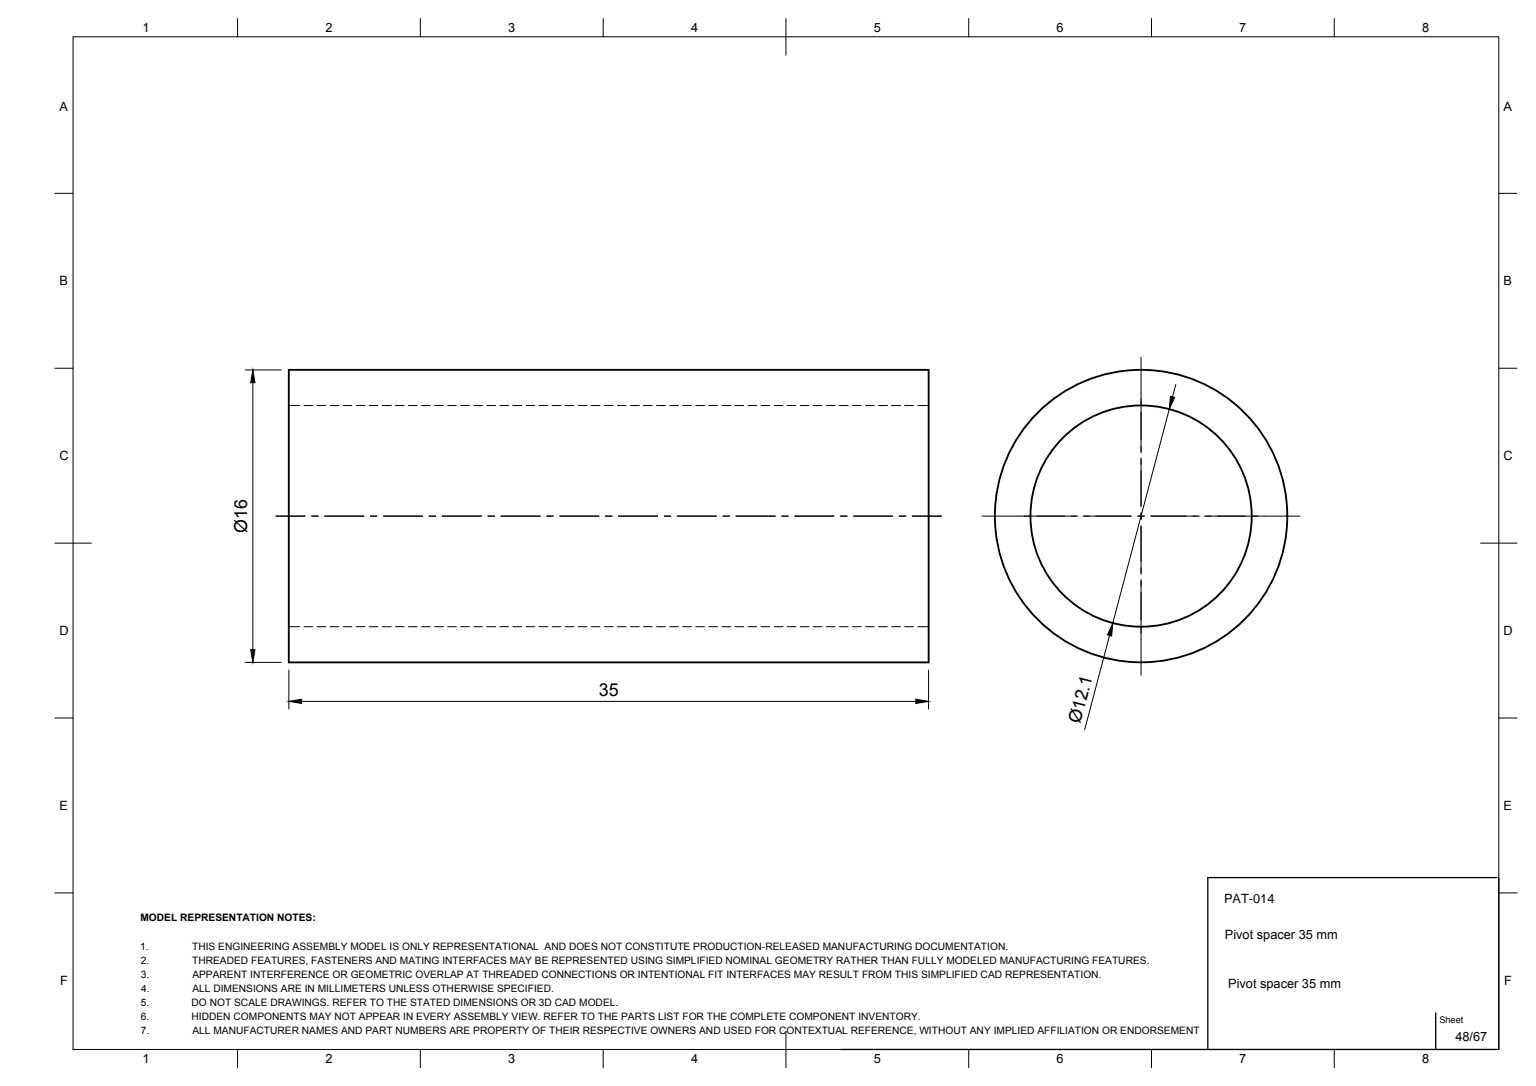
ISO-10303-21;
HEADER;
/* Generated by software containing ST-Developer
 * from STEP Tools, Inc. (www.steptools.com) 
 */

FILE_DESCRIPTION(
/* description */ ('Bin tilter linkage'),
/* implementation_level */ '2;1');

FILE_NAME(
/* name */ 'Pivot spacer 35 mm.step',
/* time_stamp */ '2026-10-28T03:26:24-07:00',
/* author */ (''),
/* organization */ (''),
/* preprocessor_version */ 'ST-DEVELOPER v20.2',
/* originating_system */ 'Autodesk Translation Framework v15.17.0.0',
/* authorisation */ '');

FILE_SCHEMA (('AUTOMOTIVE_DESIGN { 1 0 10303 214 3 1 1 }'));
ENDSEC;

DATA;
#10=MECHANICAL_DESIGN_GEOMETRIC_PRESENTATION_REPRESENTATION('',(#952),#23728);
#732=SHAPE_REPRESENTATION_RELATIONSHIP('SRR','None',#24200,#838);
#838=ADVANCED_BREP_SHAPE_REPRESENTATION('',(#1065),#23700);
#952=STYLED_ITEM('',(#24758),#1065);
#1065=MANIFOLD_SOLID_BREP('Body1',#12483);
#1422=FACE_BOUND('',#3613,.T.);
#1423=FACE_BOUND('',#3615,.T.);
#1788=PLANE('',#15055);
#1789=PLANE('',#15056);
#2498=FACE_OUTER_BOUND('',#3610,.T.);
#2499=FACE_OUTER_BOUND('',#3611,.T.);
#2500=FACE_OUTER_BOUND('',#3612,.T.);
#2501=FACE_OUTER_BOUND('',#3614,.T.);
#3610=EDGE_LOOP('',(#10651,#10652,#10653,#10654));
#3611=EDGE_LOOP('',(#10655,#10656,#10657,#10658));
#3612=EDGE_LOOP('',(#10659));
#3613=EDGE_LOOP('',(#10660));
#3614=EDGE_LOOP('',(#10661));
#3615=EDGE_LOOP('',(#10662));
#4349=LINE('',#22696,#5024);
#4350=LINE('',#22702,#5025);
#5024=VECTOR('',#18724,0.605);
#5025=VECTOR('',#18731,0.800000000000001);
#5824=CIRCLE('',#15050,0.605);
#5825=CIRCLE('',#15051,0.605);
#5826=CIRCLE('',#15053,0.800000000000001);
#5827=CIRCLE('',#15054,0.800000000000001);
#6723=VERTEX_POINT('',#22693);
#6724=VERTEX_POINT('',#22695);
#6725=VERTEX_POINT('',#22699);
#6726=VERTEX_POINT('',#22701);
#8065=EDGE_CURVE('',#6723,#6723,#5824,.T.);
#8066=EDGE_CURVE('',#6723,#6724,#4349,.T.);
#8067=EDGE_CURVE('',#6724,#6724,#5825,.T.);
#8068=EDGE_CURVE('',#6725,#6725,#5826,.T.);
#8069=EDGE_CURVE('',#6725,#6726,#4350,.T.);
#8070=EDGE_CURVE('',#6726,#6726,#5827,.T.);
#10651=ORIENTED_EDGE('',*,*,#8065,.F.);
#10652=ORIENTED_EDGE('',*,*,#8066,.T.);
#10653=ORIENTED_EDGE('',*,*,#8067,.T.);
#10654=ORIENTED_EDGE('',*,*,#8066,.F.);
#10655=ORIENTED_EDGE('',*,*,#8068,.F.);
#10656=ORIENTED_EDGE('',*,*,#8069,.T.);
#10657=ORIENTED_EDGE('',*,*,#8070,.T.);
#10658=ORIENTED_EDGE('',*,*,#8069,.F.);
#10659=ORIENTED_EDGE('',*,*,#8068,.T.);
#10660=ORIENTED_EDGE('',*,*,#8065,.T.);
#10661=ORIENTED_EDGE('',*,*,#8070,.F.);
#10662=ORIENTED_EDGE('',*,*,#8067,.F.);
#11555=CYLINDRICAL_SURFACE('',#15049,0.605);
#11556=CYLINDRICAL_SURFACE('',#15052,0.800000000000001);
#12223=ADVANCED_FACE('',(#2498),#11555,.F.);
#12224=ADVANCED_FACE('',(#2499),#11556,.T.);
#12225=ADVANCED_FACE('',(#2500,#1422),#1788,.T.);
#12226=ADVANCED_FACE('',(#2501,#1423),#1789,.F.);
#12483=CLOSED_SHELL('',(#12223,#12224,#12225,#12226));
#15048=AXIS2_PLACEMENT_3D('',#22691,#18718,#18719);
#15049=AXIS2_PLACEMENT_3D('',#22692,#18720,#18721);
#15050=AXIS2_PLACEMENT_3D('',#22694,#18722,#18723);
#15051=AXIS2_PLACEMENT_3D('',#22697,#18725,#18726);
#15052=AXIS2_PLACEMENT_3D('',#22698,#18727,#18728);
#15053=AXIS2_PLACEMENT_3D('',#22700,#18729,#18730);
#15054=AXIS2_PLACEMENT_3D('',#22703,#18732,#18733);
#15055=AXIS2_PLACEMENT_3D('',#22704,#18734,#18735);
#15056=AXIS2_PLACEMENT_3D('',#22705,#18736,#18737);
#18718=DIRECTION('axis',(0.,0.,1.));
#18719=DIRECTION('refdir',(1.,0.,0.));
#18720=DIRECTION('center_axis',(0.,1.,0.));
#18721=DIRECTION('ref_axis',(1.,0.,0.));
#18722=DIRECTION('center_axis',(0.,-1.,0.));
#18723=DIRECTION('ref_axis',(1.,0.,0.));
#18724=DIRECTION('',(0.,-1.,0.));
#18725=DIRECTION('center_axis',(0.,-1.,0.));
#18726=DIRECTION('ref_axis',(1.,0.,0.));
#18727=DIRECTION('center_axis',(0.,1.,0.));
#18728=DIRECTION('ref_axis',(1.,0.,0.));
#18729=DIRECTION('center_axis',(0.,1.,0.));
#18730=DIRECTION('ref_axis',(1.,0.,0.));
#18731=DIRECTION('',(0.,-1.,0.));
#18732=DIRECTION('center_axis',(0.,1.,0.));
#18733=DIRECTION('ref_axis',(1.,0.,0.));
#18734=DIRECTION('center_axis',(0.,1.,0.));
#18735=DIRECTION('ref_axis',(1.,0.,0.));
#18736=DIRECTION('center_axis',(0.,1.,0.));
#18737=DIRECTION('ref_axis',(1.,0.,0.));
#22691=CARTESIAN_POINT('',(0.,0.,0.));
#22692=CARTESIAN_POINT('Origin',(9.39692620785909,-4.,18.4202014332567));
#22693=CARTESIAN_POINT('',(8.79192620785908,-0.5,18.4202014332567));
#22694=CARTESIAN_POINT('Origin',(9.39692620785909,-0.5,18.4202014332567));
#22695=CARTESIAN_POINT('',(8.79192620785908,-4.,18.4202014332567));
#22696=CARTESIAN_POINT('',(8.79192620785908,-4.,18.4202014332567));
#22697=CARTESIAN_POINT('Origin',(9.39692620785909,-4.,18.4202014332567));
#22698=CARTESIAN_POINT('Origin',(9.39692620785909,-4.,18.4202014332567));
#22699=CARTESIAN_POINT('',(8.59692620785908,-0.5,18.4202014332567));
#22700=CARTESIAN_POINT('Origin',(9.39692620785909,-0.5,18.4202014332567));
#22701=CARTESIAN_POINT('',(8.59692620785908,-4.,18.4202014332567));
#22702=CARTESIAN_POINT('',(8.59692620785908,-4.,18.4202014332567));
#22703=CARTESIAN_POINT('Origin',(9.39692620785909,-4.,18.4202014332567));
#22704=CARTESIAN_POINT('Origin',(9.39692620785909,-0.5,18.4202014332567));
#22705=CARTESIAN_POINT('Origin',(9.39692620785909,-4.,18.4202014332567));
#23583=UNCERTAINTY_MEASURE_WITH_UNIT(LENGTH_MEASURE(0.001),#23729,
'DISTANCE_ACCURACY_VALUE',
'Maximum model space distance between geometric entities at asserted c
onnectivities');
#23611=UNCERTAINTY_MEASURE_WITH_UNIT(LENGTH_MEASURE(0.001),#23729,
'DISTANCE_ACCURACY_VALUE',
'Maximum model space distance between geometric entities at asserted c
onnectivities');
#23700=(
GEOMETRIC_REPRESENTATION_CONTEXT(3)
GLOBAL_UNCERTAINTY_ASSIGNED_CONTEXT((#23583))
GLOBAL_UNIT_ASSIGNED_CONTEXT((#23729,#23731,#23732))
REPRESENTATION_CONTEXT('','3D')
);
#23728=(
GEOMETRIC_REPRESENTATION_CONTEXT(3)
GLOBAL_UNCERTAINTY_ASSIGNED_CONTEXT((#23611))
GLOBAL_UNIT_ASSIGNED_CONTEXT((#23729,#23731,#23732))
REPRESENTATION_CONTEXT('','3D')
);
#23729=(
LENGTH_UNIT()
NAMED_UNIT(*)
SI_UNIT(.CENTI.,.METRE.)
);
#23731=(
NAMED_UNIT(*)
PLANE_ANGLE_UNIT()
SI_UNIT($,.RADIAN.)
);
#23732=(
NAMED_UNIT(*)
SI_UNIT($,.STERADIAN.)
SOLID_ANGLE_UNIT()
);
#23821=SHAPE_DEFINITION_REPRESENTATION(#23988,#24200);
#23988=PRODUCT_DEFINITION_SHAPE('',$,#24317);
#24200=SHAPE_REPRESENTATION('',(#15048),#23700);
#24228=PRODUCT_DEFINITION_CONTEXT('part definition',#24578,'design');
#24317=PRODUCT_DEFINITION('Pivot spacer 35 mm','Pivot spacer 35 mm',#24433,
#24228);
#24433=PRODUCT_DEFINITION_FORMATION('',$,#24668);
#24578=APPLICATION_CONTEXT(
'Core Data for Automotive Mechanical Design Process');
#24579=PRODUCT_CONTEXT('part definition',#24578,'mechanical');
#24668=PRODUCT('Pivot spacer 35 mm','Pivot spacer 35 mm',
'Pivot spacer 35 mm',(#24579));
#24752=COLOUR_RGB('Sky Blue',0.24,0.69,0.87);
#24753=FILL_AREA_STYLE_COLOUR('',#24752);
#24754=FILL_AREA_STYLE('',(#24753));
#24755=SURFACE_STYLE_FILL_AREA(#24754);
#24756=SURFACE_SIDE_STYLE('',(#24755));
#24757=SURFACE_STYLE_USAGE(.BOTH.,#24756);
#24758=PRESENTATION_STYLE_ASSIGNMENT((#24757));
ENDSEC;
END-ISO-10303-21;
